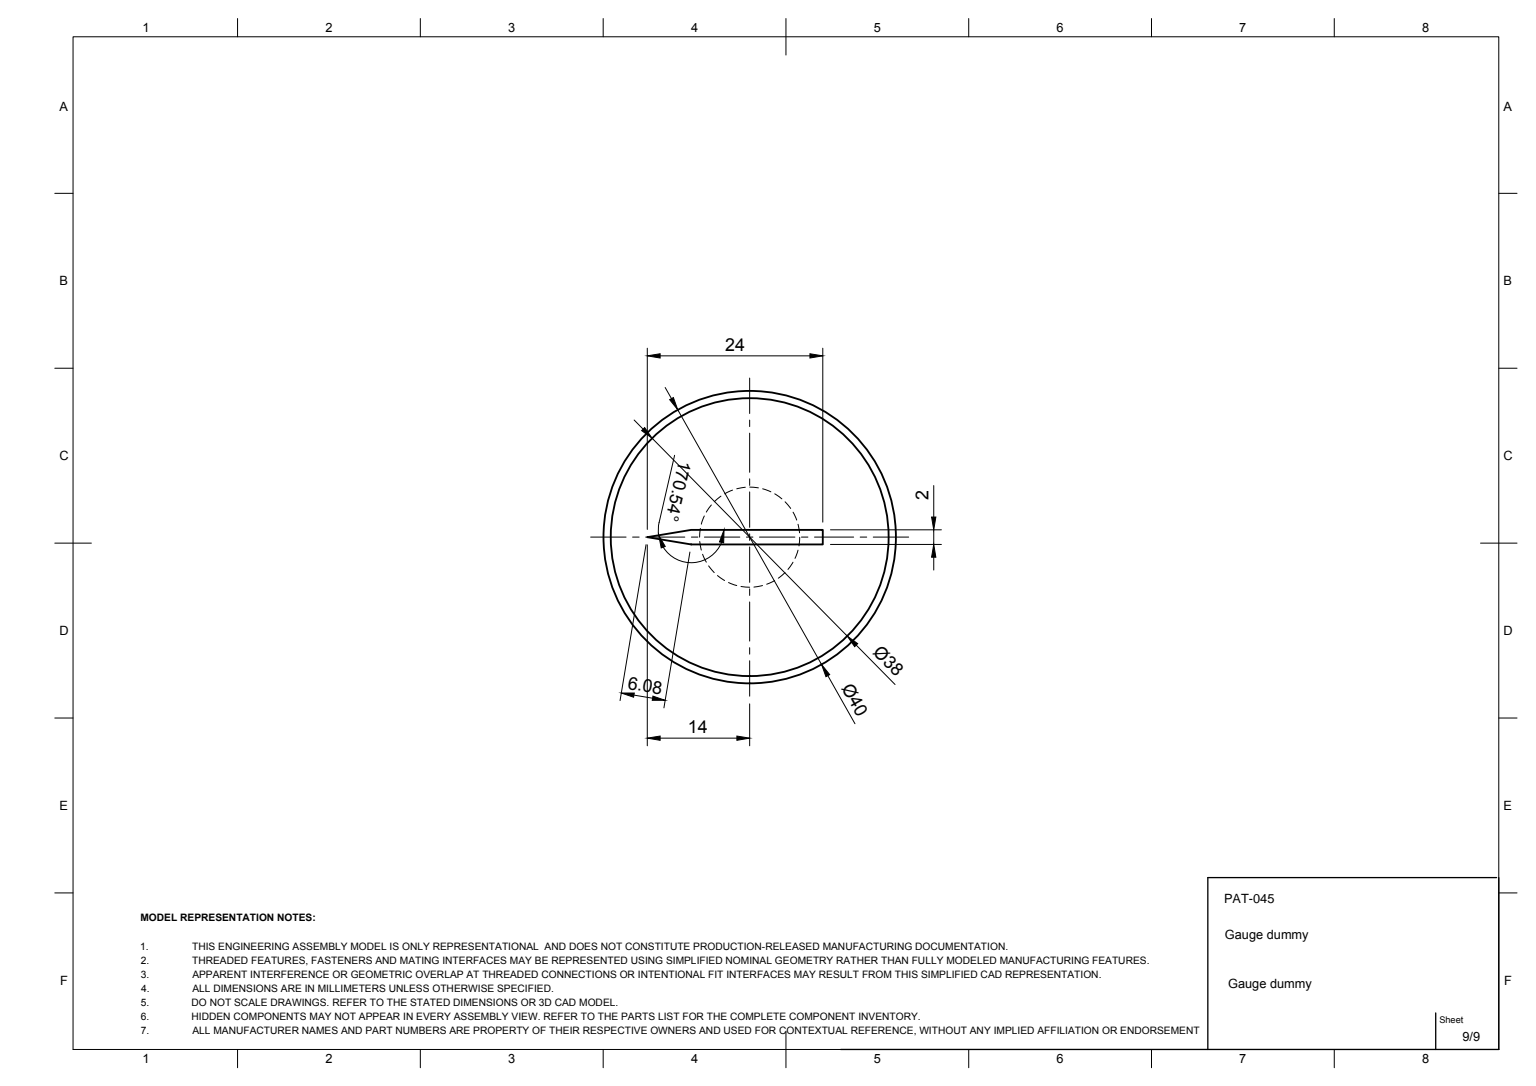
ISO-10303-21;
HEADER;
/* Generated by software containing ST-Developer
 * from STEP Tools, Inc. (www.steptools.com) 
 */

FILE_DESCRIPTION(
/* description */ ('Gauge isolation and snubber set'),
/* implementation_level */ '2;1');

FILE_NAME(
/* name */ 'Gauge dummy.step',
/* time_stamp */ '2026-10-29T16:58:15-07:00',
/* author */ (''),
/* organization */ (''),
/* preprocessor_version */ 'ST-DEVELOPER v20.2',
/* originating_system */ 'Autodesk Translation Framework v15.17.0.0',
/* authorisation */ '');

FILE_SCHEMA (('AUTOMOTIVE_DESIGN { 1 0 10303 214 3 1 1 }'));
ENDSEC;

DATA;
#10=MECHANICAL_DESIGN_GEOMETRIC_PRESENTATION_REPRESENTATION('',(#98,#99,#100),#4043);
#82=SHAPE_REPRESENTATION_RELATIONSHIP('SRR','None',#4089,#90);
#90=ADVANCED_BREP_SHAPE_REPRESENTATION('',(#108,#109,#110),#4041);
#98=STYLED_ITEM('',(#4211),#108);
#99=STYLED_ITEM('',(#4211),#109);
#100=STYLED_ITEM('',(#4211),#110);
#108=MANIFOLD_SOLID_BREP('Body1',#2215);
#109=MANIFOLD_SOLID_BREP('Off white dial',#2216);
#110=MANIFOLD_SOLID_BREP('Black pointer',#2217);
#151=FACE_BOUND('',#502,.T.);
#220=PLANE('',#2508);
#221=PLANE('',#2513);
#222=PLANE('',#2516);
#223=PLANE('',#2520);
#224=PLANE('',#2521);
#225=PLANE('',#2522);
#226=PLANE('',#2523);
#227=PLANE('',#2524);
#228=PLANE('',#2525);
#229=PLANE('',#2526);
#230=PLANE('',#2527);
#231=PLANE('',#2528);
#338=FACE_OUTER_BOUND('',#501,.T.);
#339=FACE_OUTER_BOUND('',#503,.T.);
#340=FACE_OUTER_BOUND('',#504,.T.);
#341=FACE_OUTER_BOUND('',#505,.T.);
#342=FACE_OUTER_BOUND('',#506,.T.);
#343=FACE_OUTER_BOUND('',#507,.T.);
#344=FACE_OUTER_BOUND('',#508,.T.);
#345=FACE_OUTER_BOUND('',#509,.T.);
#346=FACE_OUTER_BOUND('',#510,.T.);
#347=FACE_OUTER_BOUND('',#511,.T.);
#348=FACE_OUTER_BOUND('',#512,.T.);
#349=FACE_OUTER_BOUND('',#513,.T.);
#350=FACE_OUTER_BOUND('',#514,.T.);
#351=FACE_OUTER_BOUND('',#515,.T.);
#352=FACE_OUTER_BOUND('',#516,.T.);
#501=EDGE_LOOP('',(#1947));
#502=EDGE_LOOP('',(#1948));
#503=EDGE_LOOP('',(#1949,#1950,#1951,#1952));
#504=EDGE_LOOP('',(#1953));
#505=EDGE_LOOP('',(#1954,#1955,#1956,#1957));
#506=EDGE_LOOP('',(#1958));
#507=EDGE_LOOP('',(#1959,#1960,#1961,#1962));
#508=EDGE_LOOP('',(#1963));
#509=EDGE_LOOP('',(#1964));
#510=EDGE_LOOP('',(#1965,#1966,#1967,#1968));
#511=EDGE_LOOP('',(#1969,#1970,#1971,#1972));
#512=EDGE_LOOP('',(#1973,#1974,#1975,#1976));
#513=EDGE_LOOP('',(#1977,#1978,#1979,#1980));
#514=EDGE_LOOP('',(#1981,#1982,#1983,#1984));
#515=EDGE_LOOP('',(#1985,#1986,#1987,#1988,#1989));
#516=EDGE_LOOP('',(#1990,#1991,#1992,#1993,#1994));
#624=CIRCLE('',#2509,2.);
#625=CIRCLE('',#2510,0.685);
#626=CIRCLE('',#2512,2.);
#627=CIRCLE('',#2515,0.685);
#628=CIRCLE('',#2518,1.9);
#629=CIRCLE('',#2519,1.9);
#772=LINE('',#3895,#943);
#773=LINE('',#3901,#944);
#774=LINE('',#3907,#945);
#775=LINE('',#3914,#946);
#776=LINE('',#3916,#947);
#777=LINE('',#3918,#948);
#778=LINE('',#3919,#949);
#779=LINE('',#3922,#950);
#780=LINE('',#3924,#951);
#781=LINE('',#3925,#952);
#782=LINE('',#3928,#953);
#783=LINE('',#3930,#954);
#784=LINE('',#3931,#955);
#785=LINE('',#3934,#956);
#786=LINE('',#3936,#957);
#787=LINE('',#3937,#958);
#788=LINE('',#3939,#959);
#789=LINE('',#3940,#960);
#943=VECTOR('',#3105,2.);
#944=VECTOR('',#3114,0.685);
#945=VECTOR('',#3121,1.9);
#946=VECTOR('',#3130,1.);
#947=VECTOR('',#3131,1.);
#948=VECTOR('',#3132,1.);
#949=VECTOR('',#3133,1.);
#950=VECTOR('',#3136,1.);
#951=VECTOR('',#3137,1.);
#952=VECTOR('',#3138,1.);
#953=VECTOR('',#3141,1.);
#954=VECTOR('',#3142,1.);
#955=VECTOR('',#3143,1.);
#956=VECTOR('',#3146,1.);
#957=VECTOR('',#3147,1.);
#958=VECTOR('',#3148,1.);
#959=VECTOR('',#3151,1.);
#960=VECTOR('',#3152,1.);
#1137=VERTEX_POINT('',#3889);
#1138=VERTEX_POINT('',#3891);
#1139=VERTEX_POINT('',#3894);
#1140=VERTEX_POINT('',#3899);
#1141=VERTEX_POINT('',#3904);
#1142=VERTEX_POINT('',#3906);
#1143=VERTEX_POINT('',#3912);
#1144=VERTEX_POINT('',#3913);
#1145=VERTEX_POINT('',#3915);
#1146=VERTEX_POINT('',#3917);
#1147=VERTEX_POINT('',#3921);
#1148=VERTEX_POINT('',#3923);
#1149=VERTEX_POINT('',#3927);
#1150=VERTEX_POINT('',#3929);
#1151=VERTEX_POINT('',#3933);
#1152=VERTEX_POINT('',#3935);
#1412=EDGE_CURVE('',#1137,#1137,#624,.T.);
#1413=EDGE_CURVE('',#1138,#1138,#625,.T.);
#1414=EDGE_CURVE('',#1137,#1139,#772,.T.);
#1415=EDGE_CURVE('',#1139,#1139,#626,.T.);
#1416=EDGE_CURVE('',#1140,#1140,#627,.T.);
#1417=EDGE_CURVE('',#1140,#1138,#773,.T.);
#1418=EDGE_CURVE('',#1141,#1141,#628,.T.);
#1419=EDGE_CURVE('',#1141,#1142,#774,.T.);
#1420=EDGE_CURVE('',#1142,#1142,#629,.T.);
#1421=EDGE_CURVE('',#1143,#1144,#775,.T.);
#1422=EDGE_CURVE('',#1143,#1145,#776,.T.);
#1423=EDGE_CURVE('',#1146,#1145,#777,.T.);
#1424=EDGE_CURVE('',#1144,#1146,#778,.T.);
#1425=EDGE_CURVE('',#1144,#1147,#779,.T.);
#1426=EDGE_CURVE('',#1148,#1146,#780,.T.);
#1427=EDGE_CURVE('',#1147,#1148,#781,.T.);
#1428=EDGE_CURVE('',#1147,#1149,#782,.T.);
#1429=EDGE_CURVE('',#1150,#1148,#783,.T.);
#1430=EDGE_CURVE('',#1149,#1150,#784,.T.);
#1431=EDGE_CURVE('',#1149,#1151,#785,.T.);
#1432=EDGE_CURVE('',#1152,#1150,#786,.T.);
#1433=EDGE_CURVE('',#1151,#1152,#787,.T.);
#1434=EDGE_CURVE('',#1151,#1143,#788,.T.);
#1435=EDGE_CURVE('',#1145,#1152,#789,.T.);
#1947=ORIENTED_EDGE('',*,*,#1412,.T.);
#1948=ORIENTED_EDGE('',*,*,#1413,.F.);
#1949=ORIENTED_EDGE('',*,*,#1412,.F.);
#1950=ORIENTED_EDGE('',*,*,#1414,.T.);
#1951=ORIENTED_EDGE('',*,*,#1415,.T.);
#1952=ORIENTED_EDGE('',*,*,#1414,.F.);
#1953=ORIENTED_EDGE('',*,*,#1415,.F.);
#1954=ORIENTED_EDGE('',*,*,#1416,.F.);
#1955=ORIENTED_EDGE('',*,*,#1417,.T.);
#1956=ORIENTED_EDGE('',*,*,#1413,.T.);
#1957=ORIENTED_EDGE('',*,*,#1417,.F.);
#1958=ORIENTED_EDGE('',*,*,#1416,.T.);
#1959=ORIENTED_EDGE('',*,*,#1418,.F.);
#1960=ORIENTED_EDGE('',*,*,#1419,.T.);
#1961=ORIENTED_EDGE('',*,*,#1420,.T.);
#1962=ORIENTED_EDGE('',*,*,#1419,.F.);
#1963=ORIENTED_EDGE('',*,*,#1418,.T.);
#1964=ORIENTED_EDGE('',*,*,#1420,.F.);
#1965=ORIENTED_EDGE('',*,*,#1421,.F.);
#1966=ORIENTED_EDGE('',*,*,#1422,.T.);
#1967=ORIENTED_EDGE('',*,*,#1423,.F.);
#1968=ORIENTED_EDGE('',*,*,#1424,.F.);
#1969=ORIENTED_EDGE('',*,*,#1425,.F.);
#1970=ORIENTED_EDGE('',*,*,#1424,.T.);
#1971=ORIENTED_EDGE('',*,*,#1426,.F.);
#1972=ORIENTED_EDGE('',*,*,#1427,.F.);
#1973=ORIENTED_EDGE('',*,*,#1428,.F.);
#1974=ORIENTED_EDGE('',*,*,#1427,.T.);
#1975=ORIENTED_EDGE('',*,*,#1429,.F.);
#1976=ORIENTED_EDGE('',*,*,#1430,.F.);
#1977=ORIENTED_EDGE('',*,*,#1431,.F.);
#1978=ORIENTED_EDGE('',*,*,#1430,.T.);
#1979=ORIENTED_EDGE('',*,*,#1432,.F.);
#1980=ORIENTED_EDGE('',*,*,#1433,.F.);
#1981=ORIENTED_EDGE('',*,*,#1434,.F.);
#1982=ORIENTED_EDGE('',*,*,#1433,.T.);
#1983=ORIENTED_EDGE('',*,*,#1435,.F.);
#1984=ORIENTED_EDGE('',*,*,#1422,.F.);
#1985=ORIENTED_EDGE('',*,*,#1435,.T.);
#1986=ORIENTED_EDGE('',*,*,#1432,.T.);
#1987=ORIENTED_EDGE('',*,*,#1429,.T.);
#1988=ORIENTED_EDGE('',*,*,#1426,.T.);
#1989=ORIENTED_EDGE('',*,*,#1423,.T.);
#1990=ORIENTED_EDGE('',*,*,#1434,.T.);
#1991=ORIENTED_EDGE('',*,*,#1421,.T.);
#1992=ORIENTED_EDGE('',*,*,#1425,.T.);
#1993=ORIENTED_EDGE('',*,*,#1428,.T.);
#1994=ORIENTED_EDGE('',*,*,#1431,.T.);
#2081=CYLINDRICAL_SURFACE('',#2511,2.);
#2082=CYLINDRICAL_SURFACE('',#2514,0.685);
#2083=CYLINDRICAL_SURFACE('',#2517,1.9);
#2182=ADVANCED_FACE('',(#338,#151),#220,.T.);
#2183=ADVANCED_FACE('',(#339),#2081,.T.);
#2184=ADVANCED_FACE('',(#340),#221,.F.);
#2185=ADVANCED_FACE('',(#341),#2082,.T.);
#2186=ADVANCED_FACE('',(#342),#222,.T.);
#2187=ADVANCED_FACE('',(#343),#2083,.T.);
#2188=ADVANCED_FACE('',(#344),#223,.T.);
#2189=ADVANCED_FACE('',(#345),#224,.F.);
#2190=ADVANCED_FACE('',(#346),#225,.T.);
#2191=ADVANCED_FACE('',(#347),#226,.T.);
#2192=ADVANCED_FACE('',(#348),#227,.T.);
#2193=ADVANCED_FACE('',(#349),#228,.T.);
#2194=ADVANCED_FACE('',(#350),#229,.T.);
#2195=ADVANCED_FACE('',(#351),#230,.T.);
#2196=ADVANCED_FACE('',(#352),#231,.F.);
#2215=CLOSED_SHELL('',(#2182,#2183,#2184,#2185,#2186));
#2216=CLOSED_SHELL('',(#2187,#2188,#2189));
#2217=CLOSED_SHELL('',(#2190,#2191,#2192,#2193,#2194,#2195,#2196));
#2507=AXIS2_PLACEMENT_3D('',#3887,#3095,#3096);
#2508=AXIS2_PLACEMENT_3D('',#3888,#3097,#3098);
#2509=AXIS2_PLACEMENT_3D('',#3890,#3099,#3100);
#2510=AXIS2_PLACEMENT_3D('',#3892,#3101,#3102);
#2511=AXIS2_PLACEMENT_3D('',#3893,#3103,#3104);
#2512=AXIS2_PLACEMENT_3D('',#3896,#3106,#3107);
#2513=AXIS2_PLACEMENT_3D('',#3897,#3108,#3109);
#2514=AXIS2_PLACEMENT_3D('',#3898,#3110,#3111);
#2515=AXIS2_PLACEMENT_3D('',#3900,#3112,#3113);
#2516=AXIS2_PLACEMENT_3D('',#3902,#3115,#3116);
#2517=AXIS2_PLACEMENT_3D('',#3903,#3117,#3118);
#2518=AXIS2_PLACEMENT_3D('',#3905,#3119,#3120);
#2519=AXIS2_PLACEMENT_3D('',#3908,#3122,#3123);
#2520=AXIS2_PLACEMENT_3D('',#3909,#3124,#3125);
#2521=AXIS2_PLACEMENT_3D('',#3910,#3126,#3127);
#2522=AXIS2_PLACEMENT_3D('',#3911,#3128,#3129);
#2523=AXIS2_PLACEMENT_3D('',#3920,#3134,#3135);
#2524=AXIS2_PLACEMENT_3D('',#3926,#3139,#3140);
#2525=AXIS2_PLACEMENT_3D('',#3932,#3144,#3145);
#2526=AXIS2_PLACEMENT_3D('',#3938,#3149,#3150);
#2527=AXIS2_PLACEMENT_3D('',#3941,#3153,#3154);
#2528=AXIS2_PLACEMENT_3D('',#3942,#3155,#3156);
#3095=DIRECTION('axis',(0.,0.,1.));
#3096=DIRECTION('refdir',(1.,0.,0.));
#3097=DIRECTION('center_axis',(0.,1.,0.));
#3098=DIRECTION('ref_axis',(1.,0.,0.));
#3099=DIRECTION('center_axis',(0.,1.,0.));
#3100=DIRECTION('ref_axis',(1.,0.,0.));
#3101=DIRECTION('center_axis',(0.,1.,0.));
#3102=DIRECTION('ref_axis',(1.,0.,0.));
#3103=DIRECTION('center_axis',(0.,1.,0.));
#3104=DIRECTION('ref_axis',(1.,0.,0.));
#3105=DIRECTION('',(0.,-1.,0.));
#3106=DIRECTION('center_axis',(0.,1.,0.));
#3107=DIRECTION('ref_axis',(1.,0.,0.));
#3108=DIRECTION('center_axis',(0.,1.,0.));
#3109=DIRECTION('ref_axis',(1.,0.,0.));
#3110=DIRECTION('center_axis',(0.,1.,0.));
#3111=DIRECTION('ref_axis',(1.,0.,0.));
#3112=DIRECTION('center_axis',(0.,1.,0.));
#3113=DIRECTION('ref_axis',(1.,0.,0.));
#3114=DIRECTION('',(0.,-1.,0.));
#3115=DIRECTION('center_axis',(0.,1.,0.));
#3116=DIRECTION('ref_axis',(1.,0.,0.));
#3117=DIRECTION('center_axis',(0.,1.,0.));
#3118=DIRECTION('ref_axis',(1.,0.,0.));
#3119=DIRECTION('center_axis',(0.,1.,0.));
#3120=DIRECTION('ref_axis',(1.,0.,0.));
#3121=DIRECTION('',(0.,-1.,0.));
#3122=DIRECTION('center_axis',(0.,1.,0.));
#3123=DIRECTION('ref_axis',(1.,0.,0.));
#3124=DIRECTION('center_axis',(0.,1.,0.));
#3125=DIRECTION('ref_axis',(1.,0.,0.));
#3126=DIRECTION('center_axis',(0.,1.,0.));
#3127=DIRECTION('ref_axis',(1.,0.,0.));
#3128=DIRECTION('center_axis',(-1.,0.,0.));
#3129=DIRECTION('ref_axis',(0.,0.,1.));
#3130=DIRECTION('',(0.,0.,-1.));
#3131=DIRECTION('',(0.,1.,0.));
#3132=DIRECTION('',(0.,0.,1.));
#3133=DIRECTION('',(0.,1.,0.));
#3134=DIRECTION('center_axis',(0.,0.,-1.));
#3135=DIRECTION('ref_axis',(-1.,0.,0.));
#3136=DIRECTION('',(1.,0.,0.));
#3137=DIRECTION('',(-1.,0.,0.));
#3138=DIRECTION('',(0.,1.,0.));
#3139=DIRECTION('center_axis',(1.,0.,0.));
#3140=DIRECTION('ref_axis',(0.,0.,-1.));
#3141=DIRECTION('',(0.,0.,1.));
#3142=DIRECTION('',(0.,0.,-1.));
#3143=DIRECTION('',(0.,1.,0.));
#3144=DIRECTION('center_axis',(0.986393923832144,0.,0.164398987305357));
#3145=DIRECTION('ref_axis',(0.164398987305357,0.,-0.986393923832144));
#3146=DIRECTION('',(-0.164398987305357,0.,0.986393923832144));
#3147=DIRECTION('',(0.164398987305357,0.,-0.986393923832144));
#3148=DIRECTION('',(0.,1.,0.));
#3149=DIRECTION('center_axis',(-0.986393923832144,0.,0.164398987305357));
#3150=DIRECTION('ref_axis',(0.164398987305357,0.,0.986393923832144));
#3151=DIRECTION('',(-0.164398987305357,0.,-0.986393923832144));
#3152=DIRECTION('',(0.164398987305357,0.,0.986393923832144));
#3153=DIRECTION('center_axis',(0.,1.,0.));
#3154=DIRECTION('ref_axis',(0.,0.,1.));
#3155=DIRECTION('center_axis',(0.,1.,0.));
#3156=DIRECTION('ref_axis',(1.,0.,0.));
#3887=CARTESIAN_POINT('',(0.,0.,0.));
#3888=CARTESIAN_POINT('Origin',(0.,-5.2,2.9));
#3889=CARTESIAN_POINT('',(-2.,-5.2,2.9));
#3890=CARTESIAN_POINT('Origin',(0.,-5.2,2.9));
#3891=CARTESIAN_POINT('',(-0.685,-5.2,2.9));
#3892=CARTESIAN_POINT('Origin',(0.,-5.2,2.9));
#3893=CARTESIAN_POINT('Origin',(0.,-6.5,2.9));
#3894=CARTESIAN_POINT('',(-2.,-6.5,2.9));
#3895=CARTESIAN_POINT('',(-2.,-6.5,2.9));
#3896=CARTESIAN_POINT('Origin',(0.,-6.5,2.9));
#3897=CARTESIAN_POINT('Origin',(0.,-6.5,2.9));
#3898=CARTESIAN_POINT('Origin',(0.,-5.2,2.9));
#3899=CARTESIAN_POINT('',(-0.685,-3.6,2.9));
#3900=CARTESIAN_POINT('Origin',(0.,-3.6,2.9));
#3901=CARTESIAN_POINT('',(-0.685,-5.2,2.9));
#3902=CARTESIAN_POINT('Origin',(0.,-3.6,2.9));
#3903=CARTESIAN_POINT('Origin',(0.,-6.7,2.9));
#3904=CARTESIAN_POINT('',(-1.9,-6.5,2.9));
#3905=CARTESIAN_POINT('Origin',(0.,-6.5,2.9));
#3906=CARTESIAN_POINT('',(-1.9,-6.7,2.9));
#3907=CARTESIAN_POINT('',(-1.9,-6.7,2.9));
#3908=CARTESIAN_POINT('Origin',(0.,-6.7,2.9));
#3909=CARTESIAN_POINT('Origin',(0.,-6.5,2.9));
#3910=CARTESIAN_POINT('Origin',(0.,-6.7,2.9));
#3911=CARTESIAN_POINT('Origin',(-0.1,-6.8,1.9));
#3912=CARTESIAN_POINT('',(-0.1,-6.8,3.7));
#3913=CARTESIAN_POINT('',(-0.1,-6.8,1.9));
#3914=CARTESIAN_POINT('',(-0.1,-6.8,3.7));
#3915=CARTESIAN_POINT('',(-0.1,-6.7,3.7));
#3916=CARTESIAN_POINT('',(-0.1,-6.8,3.7));
#3917=CARTESIAN_POINT('',(-0.1,-6.7,1.9));
#3918=CARTESIAN_POINT('',(-0.1,-6.7,3.7));
#3919=CARTESIAN_POINT('',(-0.1,-6.8,1.9));
#3920=CARTESIAN_POINT('Origin',(0.1,-6.8,1.9));
#3921=CARTESIAN_POINT('',(0.1,-6.8,1.9));
#3922=CARTESIAN_POINT('',(-0.1,-6.8,1.9));
#3923=CARTESIAN_POINT('',(0.1,-6.7,1.9));
#3924=CARTESIAN_POINT('',(-0.1,-6.7,1.9));
#3925=CARTESIAN_POINT('',(0.1,-6.8,1.9));
#3926=CARTESIAN_POINT('Origin',(0.1,-6.8,3.7));
#3927=CARTESIAN_POINT('',(0.1,-6.8,3.7));
#3928=CARTESIAN_POINT('',(0.1,-6.8,1.9));
#3929=CARTESIAN_POINT('',(0.1,-6.7,3.7));
#3930=CARTESIAN_POINT('',(0.1,-6.7,1.9));
#3931=CARTESIAN_POINT('',(0.1,-6.8,3.7));
#3932=CARTESIAN_POINT('Origin',(0.,-6.8,4.3));
#3933=CARTESIAN_POINT('',(0.,-6.8,4.3));
#3934=CARTESIAN_POINT('',(0.1,-6.8,3.7));
#3935=CARTESIAN_POINT('',(0.,-6.7,4.3));
#3936=CARTESIAN_POINT('',(0.1,-6.7,3.7));
#3937=CARTESIAN_POINT('',(0.,-6.8,4.3));
#3938=CARTESIAN_POINT('Origin',(-0.1,-6.8,3.7));
#3939=CARTESIAN_POINT('',(0.,-6.8,4.3));
#3940=CARTESIAN_POINT('',(0.,-6.7,4.3));
#3941=CARTESIAN_POINT('Origin',(0.,-6.7,3.1));
#3942=CARTESIAN_POINT('Origin',(0.,-6.8,3.1));
#4030=UNCERTAINTY_MEASURE_WITH_UNIT(LENGTH_MEASURE(0.001),#4044,
'DISTANCE_ACCURACY_VALUE',
'Maximum model space distance between geometric entities at asserted c
onnectivities');
#4032=UNCERTAINTY_MEASURE_WITH_UNIT(LENGTH_MEASURE(0.001),#4044,
'DISTANCE_ACCURACY_VALUE',
'Maximum model space distance between geometric entities at asserted c
onnectivities');
#4041=(
GEOMETRIC_REPRESENTATION_CONTEXT(3)
GLOBAL_UNCERTAINTY_ASSIGNED_CONTEXT((#4030))
GLOBAL_UNIT_ASSIGNED_CONTEXT((#4044,#4046,#4047))
REPRESENTATION_CONTEXT('','3D')
);
#4043=(
GEOMETRIC_REPRESENTATION_CONTEXT(3)
GLOBAL_UNCERTAINTY_ASSIGNED_CONTEXT((#4032))
GLOBAL_UNIT_ASSIGNED_CONTEXT((#4044,#4046,#4047))
REPRESENTATION_CONTEXT('','3D')
);
#4044=(
LENGTH_UNIT()
NAMED_UNIT(*)
SI_UNIT(.CENTI.,.METRE.)
);
#4046=(
NAMED_UNIT(*)
PLANE_ANGLE_UNIT()
SI_UNIT($,.RADIAN.)
);
#4047=(
NAMED_UNIT(*)
SI_UNIT($,.STERADIAN.)
SOLID_ANGLE_UNIT()
);
#4056=SHAPE_DEFINITION_REPRESENTATION(#4066,#4089);
#4066=PRODUCT_DEFINITION_SHAPE('',$,#4100);
#4089=SHAPE_REPRESENTATION('',(#2507),#4041);
#4091=PRODUCT_DEFINITION_CONTEXT('part definition',#4123,'design');
#4100=PRODUCT_DEFINITION('Gauge dummy','Gauge dummy',#4110,#4091);
#4110=PRODUCT_DEFINITION_FORMATION('',$,#4133);
#4123=APPLICATION_CONTEXT(
'Core Data for Automotive Mechanical Design Process');
#4124=PRODUCT_CONTEXT('part definition',#4123,'mechanical');
#4133=PRODUCT('Gauge dummy','Gauge dummy','Gauge dummy',(#4124));
#4205=COLOUR_RGB('Off White',0.89,0.88,0.83);
#4206=FILL_AREA_STYLE_COLOUR('',#4205);
#4207=FILL_AREA_STYLE('',(#4206));
#4208=SURFACE_STYLE_FILL_AREA(#4207);
#4209=SURFACE_SIDE_STYLE('',(#4208));
#4210=SURFACE_STYLE_USAGE(.BOTH.,#4209);
#4211=PRESENTATION_STYLE_ASSIGNMENT((#4210));
ENDSEC;
END-ISO-10303-21;
